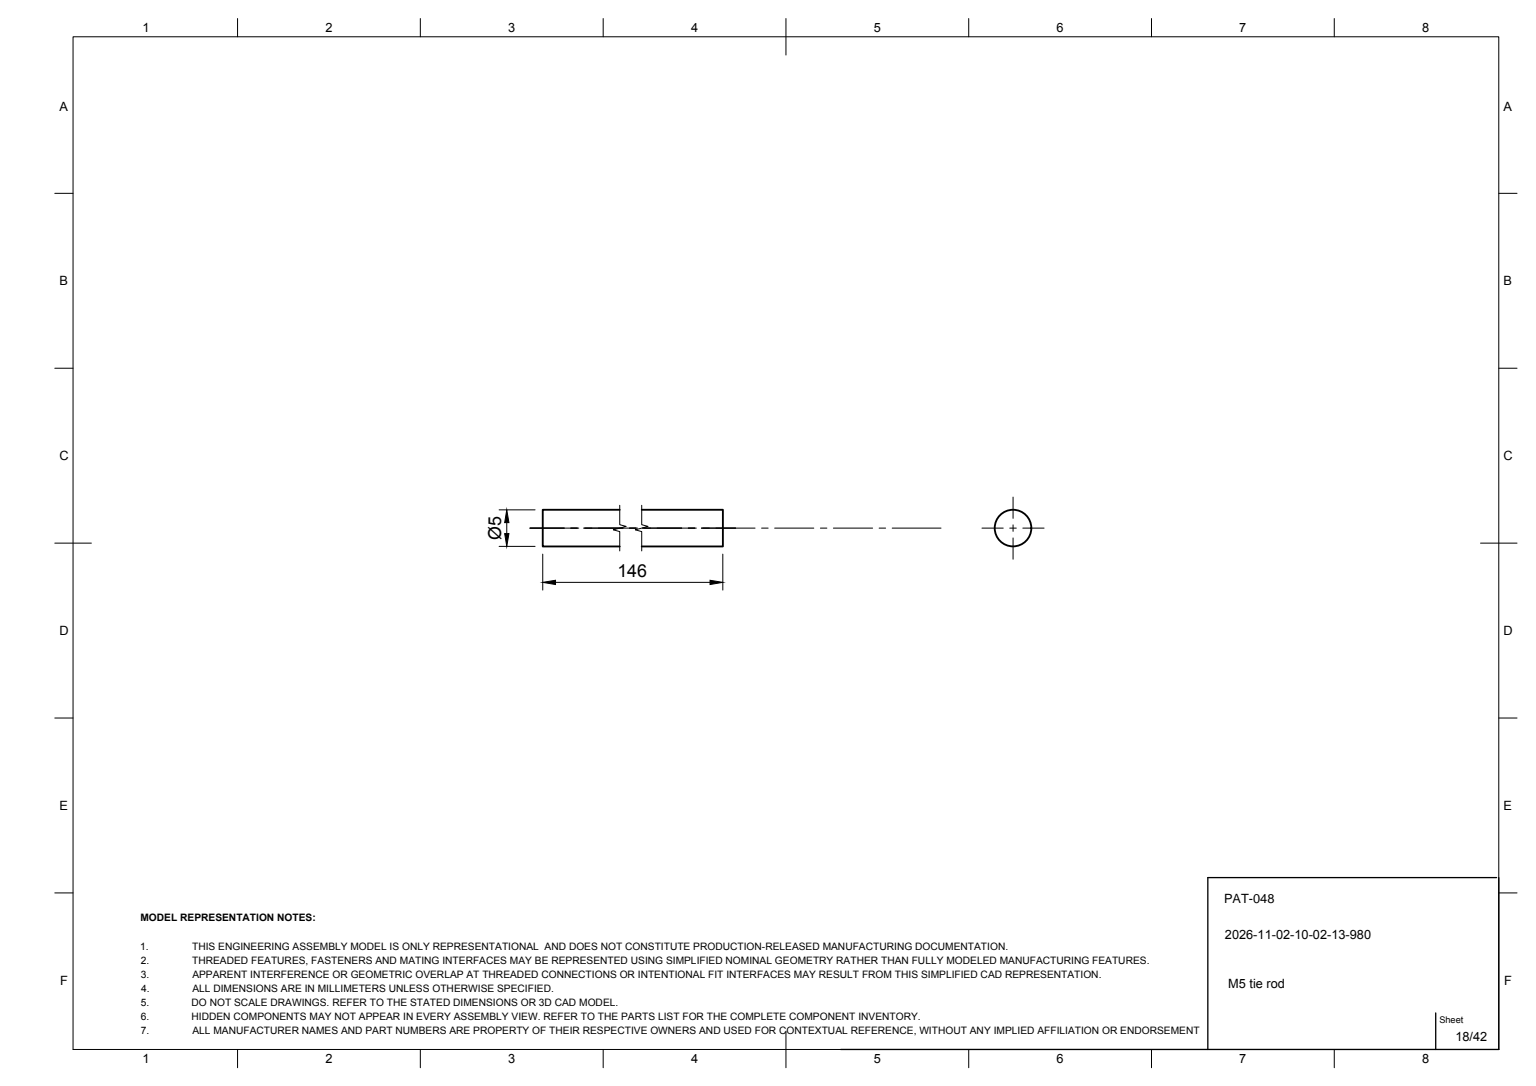
ISO-10303-21;
HEADER;
/* Generated by software containing ST-Developer
 * from STEP Tools, Inc. (www.steptools.com) 
 */

FILE_DESCRIPTION(
/* description */ ('Guided pneumatic stop gate'),
/* implementation_level */ '2;1');

FILE_NAME(
/* name */ 'M5 tie rod.step',
/* time_stamp */ '2026-10-27T21:43:45-07:00',
/* author */ (''),
/* organization */ (''),
/* preprocessor_version */ 'ST-DEVELOPER v20.2',
/* originating_system */ 'Autodesk Translation Framework v15.17.0.0',
/* authorisation */ '');

FILE_SCHEMA (('AUTOMOTIVE_DESIGN { 1 0 10303 214 3 1 1 }'));
ENDSEC;

DATA;
#10=MECHANICAL_DESIGN_GEOMETRIC_PRESENTATION_REPRESENTATION('',(#551),#14392);
#467=SHAPE_REPRESENTATION_RELATIONSHIP('SRR','None',#14602,#509);
#509=ADVANCED_BREP_SHAPE_REPRESENTATION('',(#592),#14364);
#551=STYLED_ITEM('',(#14891),#592);
#592=MANIFOLD_SOLID_BREP('Body1',#7892);
#967=PLANE('',#8796);
#968=PLANE('',#8797);
#1331=FACE_OUTER_BOUND('',#1886,.T.);
#1332=FACE_OUTER_BOUND('',#1887,.T.);
#1333=FACE_OUTER_BOUND('',#1888,.T.);
#1886=EDGE_LOOP('',(#6150,#6151,#6152,#6153));
#1887=EDGE_LOOP('',(#6154));
#1888=EDGE_LOOP('',(#6155));
#2521=LINE('',#12840,#3066);
#3066=VECTOR('',#10446,0.25);
#3528=CIRCLE('',#8794,0.25);
#3529=CIRCLE('',#8795,0.25);
#4001=VERTEX_POINT('',#12837);
#4002=VERTEX_POINT('',#12839);
#4773=EDGE_CURVE('',#4001,#4001,#3528,.T.);
#4774=EDGE_CURVE('',#4001,#4002,#2521,.T.);
#4775=EDGE_CURVE('',#4002,#4002,#3529,.T.);
#6150=ORIENTED_EDGE('',*,*,#4773,.F.);
#6151=ORIENTED_EDGE('',*,*,#4774,.T.);
#6152=ORIENTED_EDGE('',*,*,#4775,.T.);
#6153=ORIENTED_EDGE('',*,*,#4774,.F.);
#6154=ORIENTED_EDGE('',*,*,#4773,.T.);
#6155=ORIENTED_EDGE('',*,*,#4775,.F.);
#7311=CYLINDRICAL_SURFACE('',#8793,0.25);
#7613=ADVANCED_FACE('',(#1331),#7311,.T.);
#7614=ADVANCED_FACE('',(#1332),#967,.T.);
#7615=ADVANCED_FACE('',(#1333),#968,.F.);
#7892=CLOSED_SHELL('',(#7613,#7614,#7615));
#8792=AXIS2_PLACEMENT_3D('',#12835,#10440,#10441);
#8793=AXIS2_PLACEMENT_3D('',#12836,#10442,#10443);
#8794=AXIS2_PLACEMENT_3D('',#12838,#10444,#10445);
#8795=AXIS2_PLACEMENT_3D('',#12841,#10447,#10448);
#8796=AXIS2_PLACEMENT_3D('',#12842,#10449,#10450);
#8797=AXIS2_PLACEMENT_3D('',#12843,#10451,#10452);
#10440=DIRECTION('axis',(0.,0.,1.));
#10441=DIRECTION('refdir',(1.,0.,0.));
#10442=DIRECTION('center_axis',(0.,1.,0.));
#10443=DIRECTION('ref_axis',(1.,0.,0.));
#10444=DIRECTION('center_axis',(0.,1.,0.));
#10445=DIRECTION('ref_axis',(1.,0.,0.));
#10446=DIRECTION('',(0.,-1.,0.));
#10447=DIRECTION('center_axis',(0.,1.,0.));
#10448=DIRECTION('ref_axis',(1.,0.,0.));
#10449=DIRECTION('center_axis',(0.,1.,0.));
#10450=DIRECTION('ref_axis',(1.,0.,0.));
#10451=DIRECTION('center_axis',(0.,1.,0.));
#10452=DIRECTION('ref_axis',(1.,0.,0.));
#12835=CARTESIAN_POINT('',(0.,0.,0.));
#12836=CARTESIAN_POINT('Origin',(-2.,-1.,2.5));
#12837=CARTESIAN_POINT('',(-2.25,13.6,2.5));
#12838=CARTESIAN_POINT('Origin',(-2.,13.6,2.5));
#12839=CARTESIAN_POINT('',(-2.25,-1.,2.5));
#12840=CARTESIAN_POINT('',(-2.25,-1.,2.5));
#12841=CARTESIAN_POINT('Origin',(-2.,-1.,2.5));
#12842=CARTESIAN_POINT('Origin',(-2.,13.6,2.5));
#12843=CARTESIAN_POINT('Origin',(-2.,-1.,2.5));
#14316=UNCERTAINTY_MEASURE_WITH_UNIT(LENGTH_MEASURE(0.001),#14393,
'DISTANCE_ACCURACY_VALUE',
'Maximum model space distance between geometric entities at asserted c
onnectivities');
#14344=UNCERTAINTY_MEASURE_WITH_UNIT(LENGTH_MEASURE(0.001),#14393,
'DISTANCE_ACCURACY_VALUE',
'Maximum model space distance between geometric entities at asserted c
onnectivities');
#14364=(
GEOMETRIC_REPRESENTATION_CONTEXT(3)
GLOBAL_UNCERTAINTY_ASSIGNED_CONTEXT((#14316))
GLOBAL_UNIT_ASSIGNED_CONTEXT((#14393,#14395,#14396))
REPRESENTATION_CONTEXT('','3D')
);
#14392=(
GEOMETRIC_REPRESENTATION_CONTEXT(3)
GLOBAL_UNCERTAINTY_ASSIGNED_CONTEXT((#14344))
GLOBAL_UNIT_ASSIGNED_CONTEXT((#14393,#14395,#14396))
REPRESENTATION_CONTEXT('','3D')
);
#14393=(
LENGTH_UNIT()
NAMED_UNIT(*)
SI_UNIT(.CENTI.,.METRE.)
);
#14395=(
NAMED_UNIT(*)
PLANE_ANGLE_UNIT()
SI_UNIT($,.RADIAN.)
);
#14396=(
NAMED_UNIT(*)
SI_UNIT($,.STERADIAN.)
SOLID_ANGLE_UNIT()
);
#14416=SHAPE_DEFINITION_REPRESENTATION(#14465,#14602);
#14465=PRODUCT_DEFINITION_SHAPE('',$,#14650);
#14602=SHAPE_REPRESENTATION('',(#8792),#14364);
#14630=PRODUCT_DEFINITION_CONTEXT('part definition',#14773,'design');
#14650=PRODUCT_DEFINITION('M5 tie rod','M5 tie rod',#14697,#14630);
#14697=PRODUCT_DEFINITION_FORMATION('',$,#14794);
#14773=APPLICATION_CONTEXT(
'Core Data for Automotive Mechanical Design Process');
#14774=PRODUCT_CONTEXT('part definition',#14773,'mechanical');
#14794=PRODUCT('M5 tie rod','M5 tie rod','M5 tie rod',(#14774));
#14885=COLOUR_RGB('Grey',0.48,0.52,0.57);
#14886=FILL_AREA_STYLE_COLOUR('',#14885);
#14887=FILL_AREA_STYLE('',(#14886));
#14888=SURFACE_STYLE_FILL_AREA(#14887);
#14889=SURFACE_SIDE_STYLE('',(#14888));
#14890=SURFACE_STYLE_USAGE(.BOTH.,#14889);
#14891=PRESENTATION_STYLE_ASSIGNMENT((#14890));
ENDSEC;
END-ISO-10303-21;
